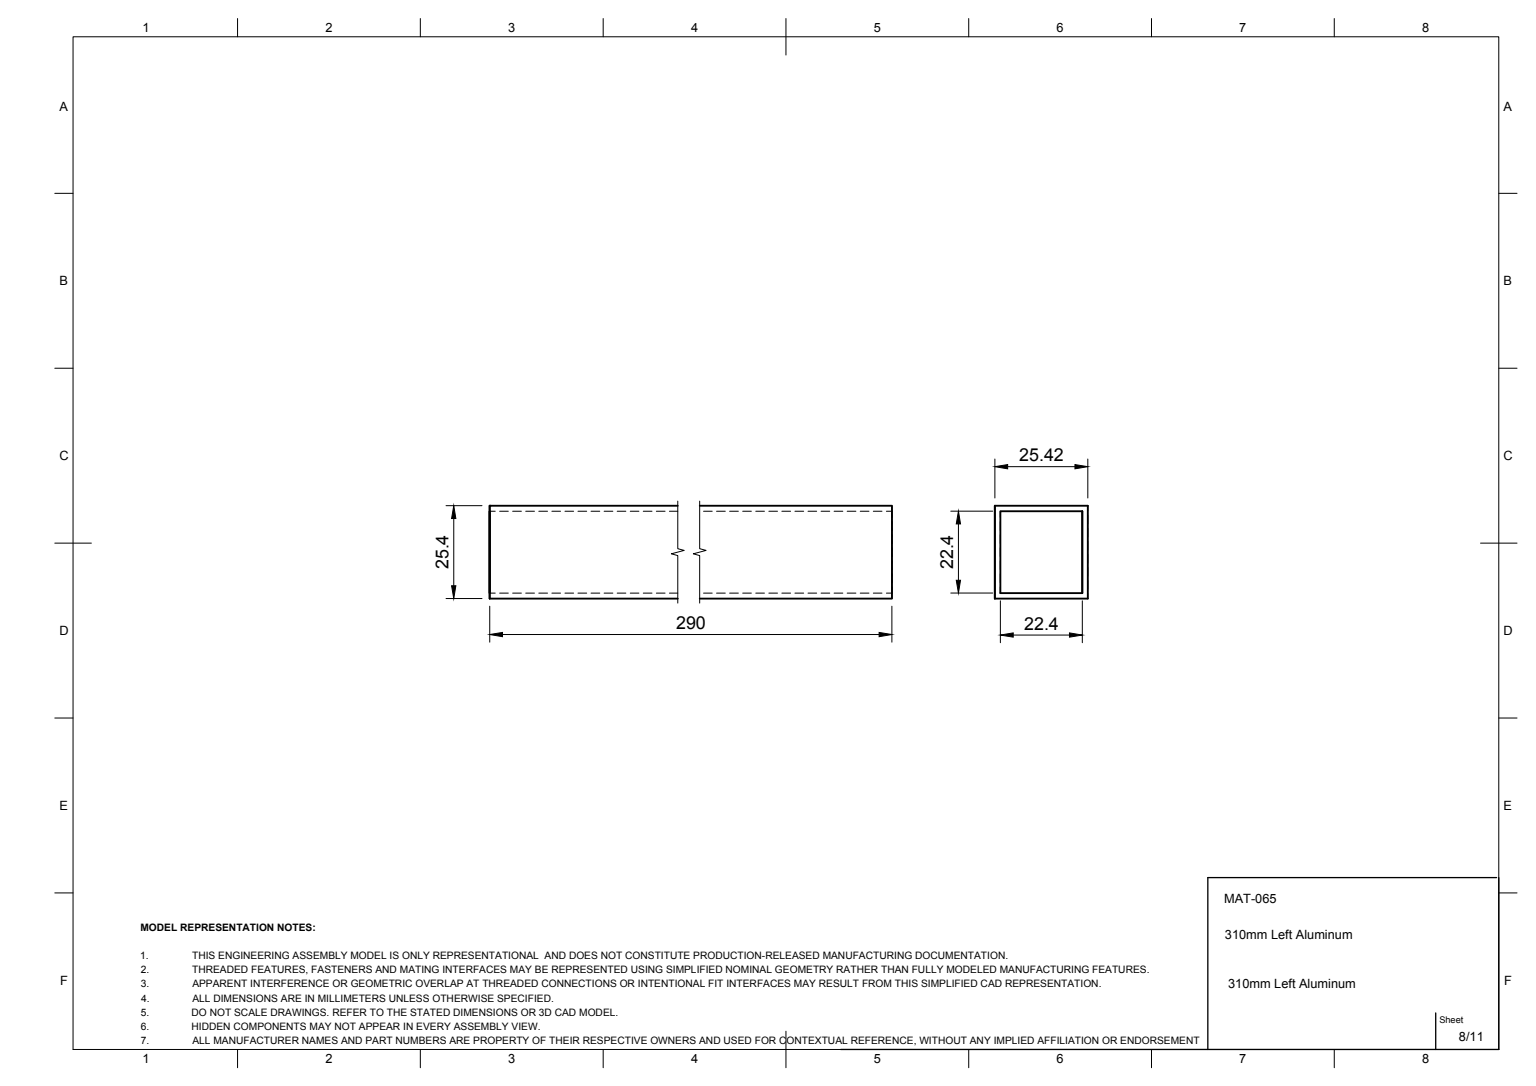
ISO-10303-21;
HEADER;
/* Generated by software containing ST-Developer
 * from STEP Tools, Inc. (www.steptools.com) 
 */

FILE_DESCRIPTION(
/* description */ (
'CAx-IF Rec.Pracs.---Representation and Presentation of Product Manufa
cturing Information (PMI)---4.0---2014-10-13'),
/* implementation_level */ '2;1');

FILE_NAME(
/* name */ '310mm Left Aluminum.step',
/* time_stamp */ '2026-11-15T23:28:27-08:00',
/* author */ (''),
/* organization */ (''),
/* preprocessor_version */ 'ST-DEVELOPER v20.2',
/* originating_system */ 'Autodesk Translation Framework v15.17.0.0',
/* authorisation */ '');

FILE_SCHEMA (('AUTOMOTIVE_DESIGN { 1 0 10303 214 3 1 1 }'));
ENDSEC;

DATA;
#10=MECHANICAL_DESIGN_GEOMETRIC_PRESENTATION_REPRESENTATION('',(#193),#7756);
#175=SHAPE_REPRESENTATION_RELATIONSHIP('SRR','None',#7823,#184);
#184=ADVANCED_BREP_SHAPE_REPRESENTATION('',(#202),#7751);
#193=STYLED_ITEM('',(#7877),#202);
#202=MANIFOLD_SOLID_BREP('Body1',#4630);
#405=FACE_BOUND('',#775,.T.);
#406=FACE_BOUND('',#777,.T.);
#506=FACE_OUTER_BOUND('',#766,.T.);
#507=FACE_OUTER_BOUND('',#767,.T.);
#508=FACE_OUTER_BOUND('',#768,.T.);
#509=FACE_OUTER_BOUND('',#769,.T.);
#510=FACE_OUTER_BOUND('',#770,.T.);
#511=FACE_OUTER_BOUND('',#771,.T.);
#512=FACE_OUTER_BOUND('',#772,.T.);
#513=FACE_OUTER_BOUND('',#773,.T.);
#514=FACE_OUTER_BOUND('',#774,.T.);
#515=FACE_OUTER_BOUND('',#776,.T.);
#766=EDGE_LOOP('',(#3263,#3264,#3265,#3266));
#767=EDGE_LOOP('',(#3267,#3268,#3269,#3270));
#768=EDGE_LOOP('',(#3271,#3272,#3273,#3274));
#769=EDGE_LOOP('',(#3275,#3276,#3277,#3278));
#770=EDGE_LOOP('',(#3279,#3280,#3281,#3282));
#771=EDGE_LOOP('',(#3283,#3284,#3285,#3286));
#772=EDGE_LOOP('',(#3287,#3288,#3289,#3290));
#773=EDGE_LOOP('',(#3291,#3292,#3293,#3294));
#774=EDGE_LOOP('',(#3295,#3296,#3297,#3298));
#775=EDGE_LOOP('',(#3299,#3300,#3301,#3302));
#776=EDGE_LOOP('',(#3303,#3304,#3305,#3306));
#777=EDGE_LOOP('',(#3307,#3308,#3309,#3310));
#1101=LINE('',#6707,#1594);
#1102=LINE('',#6709,#1595);
#1103=LINE('',#6711,#1596);
#1104=LINE('',#6712,#1597);
#1105=LINE('',#6715,#1598);
#1106=LINE('',#6717,#1599);
#1107=LINE('',#6718,#1600);
#1108=LINE('',#6721,#1601);
#1109=LINE('',#6723,#1602);
#1110=LINE('',#6724,#1603);
#1111=LINE('',#6728,#1604);
#1112=LINE('',#6730,#1605);
#1113=LINE('',#6732,#1606);
#1114=LINE('',#6733,#1607);
#1115=LINE('',#6736,#1608);
#1116=LINE('',#6738,#1609);
#1117=LINE('',#6739,#1610);
#1118=LINE('',#6742,#1611);
#1119=LINE('',#6744,#1612);
#1120=LINE('',#6745,#1613);
#1121=LINE('',#6747,#1614);
#1122=LINE('',#6748,#1615);
#1123=LINE('',#6750,#1616);
#1124=LINE('',#6751,#1617);
#1594=VECTOR('',#5415,1.);
#1595=VECTOR('',#5416,1.);
#1596=VECTOR('',#5417,1.);
#1597=VECTOR('',#5418,1.);
#1598=VECTOR('',#5421,1.);
#1599=VECTOR('',#5422,1.);
#1600=VECTOR('',#5423,1.);
#1601=VECTOR('',#5426,1.);
#1602=VECTOR('',#5427,1.);
#1603=VECTOR('',#5428,1.);
#1604=VECTOR('',#5431,1.);
#1605=VECTOR('',#5432,1.);
#1606=VECTOR('',#5433,1.);
#1607=VECTOR('',#5434,1.);
#1608=VECTOR('',#5437,1.);
#1609=VECTOR('',#5438,1.);
#1610=VECTOR('',#5439,1.);
#1611=VECTOR('',#5442,1.);
#1612=VECTOR('',#5443,1.);
#1613=VECTOR('',#5444,1.);
#1614=VECTOR('',#5447,1.);
#1615=VECTOR('',#5448,1.);
#1616=VECTOR('',#5451,1.);
#1617=VECTOR('',#5452,1.);
#2068=VERTEX_POINT('',#6705);
#2069=VERTEX_POINT('',#6706);
#2070=VERTEX_POINT('',#6708);
#2071=VERTEX_POINT('',#6710);
#2072=VERTEX_POINT('',#6714);
#2073=VERTEX_POINT('',#6716);
#2074=VERTEX_POINT('',#6720);
#2075=VERTEX_POINT('',#6722);
#2076=VERTEX_POINT('',#6726);
#2077=VERTEX_POINT('',#6727);
#2078=VERTEX_POINT('',#6729);
#2079=VERTEX_POINT('',#6731);
#2080=VERTEX_POINT('',#6735);
#2081=VERTEX_POINT('',#6737);
#2082=VERTEX_POINT('',#6741);
#2083=VERTEX_POINT('',#6743);
#2515=EDGE_CURVE('',#2068,#2069,#1101,.T.);
#2516=EDGE_CURVE('',#2070,#2068,#1102,.T.);
#2517=EDGE_CURVE('',#2070,#2071,#1103,.T.);
#2518=EDGE_CURVE('',#2071,#2069,#1104,.T.);
#2519=EDGE_CURVE('',#2068,#2072,#1105,.T.);
#2520=EDGE_CURVE('',#2073,#2072,#1106,.T.);
#2521=EDGE_CURVE('',#2070,#2073,#1107,.T.);
#2522=EDGE_CURVE('',#2072,#2074,#1108,.T.);
#2523=EDGE_CURVE('',#2075,#2074,#1109,.T.);
#2524=EDGE_CURVE('',#2073,#2075,#1110,.T.);
#2525=EDGE_CURVE('',#2076,#2077,#1111,.T.);
#2526=EDGE_CURVE('',#2078,#2076,#1112,.T.);
#2527=EDGE_CURVE('',#2078,#2079,#1113,.T.);
#2528=EDGE_CURVE('',#2079,#2077,#1114,.T.);
#2529=EDGE_CURVE('',#2076,#2080,#1115,.T.);
#2530=EDGE_CURVE('',#2081,#2080,#1116,.T.);
#2531=EDGE_CURVE('',#2078,#2081,#1117,.T.);
#2532=EDGE_CURVE('',#2080,#2082,#1118,.T.);
#2533=EDGE_CURVE('',#2083,#2082,#1119,.T.);
#2534=EDGE_CURVE('',#2081,#2083,#1120,.T.);
#2535=EDGE_CURVE('',#2077,#2082,#1121,.T.);
#2536=EDGE_CURVE('',#2079,#2083,#1122,.T.);
#2537=EDGE_CURVE('',#2069,#2074,#1123,.T.);
#2538=EDGE_CURVE('',#2071,#2075,#1124,.T.);
#3263=ORIENTED_EDGE('',*,*,#2515,.F.);
#3264=ORIENTED_EDGE('',*,*,#2516,.F.);
#3265=ORIENTED_EDGE('',*,*,#2517,.T.);
#3266=ORIENTED_EDGE('',*,*,#2518,.T.);
#3267=ORIENTED_EDGE('',*,*,#2519,.T.);
#3268=ORIENTED_EDGE('',*,*,#2520,.F.);
#3269=ORIENTED_EDGE('',*,*,#2521,.F.);
#3270=ORIENTED_EDGE('',*,*,#2516,.T.);
#3271=ORIENTED_EDGE('',*,*,#2522,.T.);
#3272=ORIENTED_EDGE('',*,*,#2523,.F.);
#3273=ORIENTED_EDGE('',*,*,#2524,.F.);
#3274=ORIENTED_EDGE('',*,*,#2520,.T.);
#3275=ORIENTED_EDGE('',*,*,#2525,.F.);
#3276=ORIENTED_EDGE('',*,*,#2526,.F.);
#3277=ORIENTED_EDGE('',*,*,#2527,.T.);
#3278=ORIENTED_EDGE('',*,*,#2528,.T.);
#3279=ORIENTED_EDGE('',*,*,#2529,.T.);
#3280=ORIENTED_EDGE('',*,*,#2530,.F.);
#3281=ORIENTED_EDGE('',*,*,#2531,.F.);
#3282=ORIENTED_EDGE('',*,*,#2526,.T.);
#3283=ORIENTED_EDGE('',*,*,#2532,.T.);
#3284=ORIENTED_EDGE('',*,*,#2533,.F.);
#3285=ORIENTED_EDGE('',*,*,#2534,.F.);
#3286=ORIENTED_EDGE('',*,*,#2530,.T.);
#3287=ORIENTED_EDGE('',*,*,#2535,.F.);
#3288=ORIENTED_EDGE('',*,*,#2528,.F.);
#3289=ORIENTED_EDGE('',*,*,#2536,.T.);
#3290=ORIENTED_EDGE('',*,*,#2533,.T.);
#3291=ORIENTED_EDGE('',*,*,#2537,.F.);
#3292=ORIENTED_EDGE('',*,*,#2518,.F.);
#3293=ORIENTED_EDGE('',*,*,#2538,.T.);
#3294=ORIENTED_EDGE('',*,*,#2523,.T.);
#3295=ORIENTED_EDGE('',*,*,#2517,.F.);
#3296=ORIENTED_EDGE('',*,*,#2521,.T.);
#3297=ORIENTED_EDGE('',*,*,#2524,.T.);
#3298=ORIENTED_EDGE('',*,*,#2538,.F.);
#3299=ORIENTED_EDGE('',*,*,#2527,.F.);
#3300=ORIENTED_EDGE('',*,*,#2531,.T.);
#3301=ORIENTED_EDGE('',*,*,#2534,.T.);
#3302=ORIENTED_EDGE('',*,*,#2536,.F.);
#3303=ORIENTED_EDGE('',*,*,#2515,.T.);
#3304=ORIENTED_EDGE('',*,*,#2537,.T.);
#3305=ORIENTED_EDGE('',*,*,#2522,.F.);
#3306=ORIENTED_EDGE('',*,*,#2519,.F.);
#3307=ORIENTED_EDGE('',*,*,#2525,.T.);
#3308=ORIENTED_EDGE('',*,*,#2535,.T.);
#3309=ORIENTED_EDGE('',*,*,#2532,.F.);
#3310=ORIENTED_EDGE('',*,*,#2529,.F.);
#4260=PLANE('',#4821);
#4261=PLANE('',#4822);
#4262=PLANE('',#4823);
#4263=PLANE('',#4824);
#4264=PLANE('',#4825);
#4265=PLANE('',#4826);
#4266=PLANE('',#4827);
#4267=PLANE('',#4828);
#4268=PLANE('',#4829);
#4269=PLANE('',#4830);
#4447=ADVANCED_FACE('',(#506),#4260,.T.);
#4448=ADVANCED_FACE('',(#507),#4261,.F.);
#4449=ADVANCED_FACE('',(#508),#4262,.F.);
#4450=ADVANCED_FACE('',(#509),#4263,.T.);
#4451=ADVANCED_FACE('',(#510),#4264,.F.);
#4452=ADVANCED_FACE('',(#511),#4265,.F.);
#4453=ADVANCED_FACE('',(#512),#4266,.T.);
#4454=ADVANCED_FACE('',(#513),#4267,.T.);
#4455=ADVANCED_FACE('',(#514,#405),#4268,.T.);
#4456=ADVANCED_FACE('',(#515,#406),#4269,.F.);
#4630=CLOSED_SHELL('',(#4447,#4448,#4449,#4450,#4451,#4452,#4453,#4454,
#4455,#4456));
#4820=AXIS2_PLACEMENT_3D('',#6703,#5411,#5412);
#4821=AXIS2_PLACEMENT_3D('',#6704,#5413,#5414);
#4822=AXIS2_PLACEMENT_3D('',#6713,#5419,#5420);
#4823=AXIS2_PLACEMENT_3D('',#6719,#5424,#5425);
#4824=AXIS2_PLACEMENT_3D('',#6725,#5429,#5430);
#4825=AXIS2_PLACEMENT_3D('',#6734,#5435,#5436);
#4826=AXIS2_PLACEMENT_3D('',#6740,#5440,#5441);
#4827=AXIS2_PLACEMENT_3D('',#6746,#5445,#5446);
#4828=AXIS2_PLACEMENT_3D('',#6749,#5449,#5450);
#4829=AXIS2_PLACEMENT_3D('',#6752,#5453,#5454);
#4830=AXIS2_PLACEMENT_3D('',#6753,#5455,#5456);
#5411=DIRECTION('axis',(0.,0.,1.));
#5412=DIRECTION('refdir',(1.,0.,0.));
#5413=DIRECTION('center_axis',(0.,1.,0.));
#5414=DIRECTION('ref_axis',(0.,0.,1.));
#5415=DIRECTION('',(1.,0.,0.));
#5416=DIRECTION('',(0.,0.,-1.));
#5417=DIRECTION('',(1.,0.,0.));
#5418=DIRECTION('',(0.,0.,-1.));
#5419=DIRECTION('center_axis',(1.,0.,0.));
#5420=DIRECTION('ref_axis',(0.,0.,-1.));
#5421=DIRECTION('',(0.,-1.,0.));
#5422=DIRECTION('',(0.,0.,-1.));
#5423=DIRECTION('',(0.,-1.,0.));
#5424=DIRECTION('center_axis',(0.,1.,0.));
#5425=DIRECTION('ref_axis',(0.,0.,1.));
#5426=DIRECTION('',(1.,0.,0.));
#5427=DIRECTION('',(0.,0.,-1.));
#5428=DIRECTION('',(1.,0.,0.));
#5429=DIRECTION('center_axis',(1.,0.,0.));
#5430=DIRECTION('ref_axis',(0.,0.,-1.));
#5431=DIRECTION('',(0.,-1.,0.));
#5432=DIRECTION('',(0.,0.,-1.));
#5433=DIRECTION('',(0.,-1.,0.));
#5434=DIRECTION('',(0.,0.,-1.));
#5435=DIRECTION('center_axis',(0.,1.,0.));
#5436=DIRECTION('ref_axis',(0.,0.,1.));
#5437=DIRECTION('',(1.,0.,0.));
#5438=DIRECTION('',(0.,0.,-1.));
#5439=DIRECTION('',(1.,0.,0.));
#5440=DIRECTION('center_axis',(1.,0.,0.));
#5441=DIRECTION('ref_axis',(0.,0.,-1.));
#5442=DIRECTION('',(0.,-1.,0.));
#5443=DIRECTION('',(0.,0.,-1.));
#5444=DIRECTION('',(0.,-1.,0.));
#5445=DIRECTION('center_axis',(0.,1.,0.));
#5446=DIRECTION('ref_axis',(0.,0.,1.));
#5447=DIRECTION('',(1.,0.,0.));
#5448=DIRECTION('',(1.,0.,0.));
#5449=DIRECTION('center_axis',(1.,0.,0.));
#5450=DIRECTION('ref_axis',(0.,0.,-1.));
#5451=DIRECTION('',(0.,-1.,0.));
#5452=DIRECTION('',(0.,-1.,0.));
#5453=DIRECTION('center_axis',(0.,0.,1.));
#5454=DIRECTION('ref_axis',(1.,0.,0.));
#5455=DIRECTION('center_axis',(0.,0.,1.));
#5456=DIRECTION('ref_axis',(1.,0.,0.));
#6703=CARTESIAN_POINT('',(0.,0.,0.));
#6704=CARTESIAN_POINT('Origin',(-0.0489786583930254,0.0564453285901962,
0.29));
#6705=CARTESIAN_POINT('',(-0.0616786583930254,0.0564453285901962,0.));
#6706=CARTESIAN_POINT('',(-0.0362786583930254,0.0564453285901962,0.));
#6707=CARTESIAN_POINT('',(-0.0489786583930254,0.0564453285901962,0.));
#6708=CARTESIAN_POINT('',(-0.0616786583930254,0.0564453285901962,0.29));
#6709=CARTESIAN_POINT('',(-0.0616786583930254,0.0564453285901962,0.29));
#6710=CARTESIAN_POINT('',(-0.0362786583930254,0.0564453285901962,0.29));
#6711=CARTESIAN_POINT('',(-0.0489786583930254,0.0564453285901962,0.29));
#6712=CARTESIAN_POINT('',(-0.0362786583930254,0.0564453285901962,0.29));
#6713=CARTESIAN_POINT('Origin',(-0.0616786583930254,0.0437453285901962,
0.29));
#6714=CARTESIAN_POINT('',(-0.0616786583930254,0.0310453285901962,0.));
#6715=CARTESIAN_POINT('',(-0.0616786583930254,0.0437453285901962,0.));
#6716=CARTESIAN_POINT('',(-0.0616786583930254,0.0310453285901962,0.29));
#6717=CARTESIAN_POINT('',(-0.0616786583930254,0.0310453285901962,0.29));
#6718=CARTESIAN_POINT('',(-0.0616786583930254,0.0437453285901962,0.29));
#6719=CARTESIAN_POINT('Origin',(-0.0489786583930254,0.0310453285901962,
0.29));
#6720=CARTESIAN_POINT('',(-0.0362786583930254,0.0310453285901962,0.));
#6721=CARTESIAN_POINT('',(-0.0489786583930254,0.0310453285901962,0.));
#6722=CARTESIAN_POINT('',(-0.0362786583930254,0.0310453285901962,0.29));
#6723=CARTESIAN_POINT('',(-0.0362786583930254,0.0310453285901962,0.29));
#6724=CARTESIAN_POINT('',(-0.0489786583930254,0.0310453285901962,0.29));
#6725=CARTESIAN_POINT('Origin',(-0.0601786583930254,0.0437453285901962,
0.29));
#6726=CARTESIAN_POINT('',(-0.0601786583930254,0.0549453285901962,0.));
#6727=CARTESIAN_POINT('',(-0.0601786583930254,0.0325453285901962,0.));
#6728=CARTESIAN_POINT('',(-0.0601786583930254,0.0437453285901962,0.));
#6729=CARTESIAN_POINT('',(-0.0601786583930254,0.0549453285901962,0.29));
#6730=CARTESIAN_POINT('',(-0.0601786583930254,0.0549453285901962,0.29));
#6731=CARTESIAN_POINT('',(-0.0601786583930254,0.0325453285901962,0.29));
#6732=CARTESIAN_POINT('',(-0.0601786583930254,0.0437453285901962,0.29));
#6733=CARTESIAN_POINT('',(-0.0601786583930254,0.0325453285901962,0.29));
#6734=CARTESIAN_POINT('Origin',(-0.0489786583930254,0.0549453285901962,
0.29));
#6735=CARTESIAN_POINT('',(-0.0377786583930254,0.0549453285901962,0.));
#6736=CARTESIAN_POINT('',(-0.0489786583930254,0.0549453285901962,0.));
#6737=CARTESIAN_POINT('',(-0.0377786583930254,0.0549453285901962,0.29));
#6738=CARTESIAN_POINT('',(-0.0377786583930254,0.0549453285901962,0.29));
#6739=CARTESIAN_POINT('',(-0.0489786583930254,0.0549453285901962,0.29));
#6740=CARTESIAN_POINT('Origin',(-0.0377786583930254,0.0437453285901962,
0.29));
#6741=CARTESIAN_POINT('',(-0.0377786583930254,0.0325453285901962,0.));
#6742=CARTESIAN_POINT('',(-0.0377786583930254,0.0437453285901962,0.));
#6743=CARTESIAN_POINT('',(-0.0377786583930254,0.0325453285901962,0.29));
#6744=CARTESIAN_POINT('',(-0.0377786583930254,0.0325453285901962,0.29));
#6745=CARTESIAN_POINT('',(-0.0377786583930254,0.0437453285901962,0.29));
#6746=CARTESIAN_POINT('Origin',(-0.0489786583930254,0.0325453285901962,
0.29));
#6747=CARTESIAN_POINT('',(-0.0489786583930254,0.0325453285901962,0.));
#6748=CARTESIAN_POINT('',(-0.0489786583930254,0.0325453285901962,0.29));
#6749=CARTESIAN_POINT('Origin',(-0.0362786583930254,0.0437453285901962,
0.29));
#6750=CARTESIAN_POINT('',(-0.0362786583930254,0.0437453285901962,0.));
#6751=CARTESIAN_POINT('',(-0.0362786583930254,0.0437453285901962,0.29));
#6752=CARTESIAN_POINT('Origin',(-0.0489786583930254,0.0437453285901962,
0.29));
#6753=CARTESIAN_POINT('Origin',(-0.0489786583930254,0.0437453285901962,
0.));
#7740=UNCERTAINTY_MEASURE_WITH_UNIT(LENGTH_MEASURE(1.E-5),#7757,
'DISTANCE_ACCURACY_VALUE',
'Maximum model space distance between geometric entities at asserted c
onnectivities');
#7745=UNCERTAINTY_MEASURE_WITH_UNIT(LENGTH_MEASURE(1.E-5),#7757,
'DISTANCE_ACCURACY_VALUE',
'Maximum model space distance between geometric entities at asserted c
onnectivities');
#7751=(
GEOMETRIC_REPRESENTATION_CONTEXT(3)
GLOBAL_UNCERTAINTY_ASSIGNED_CONTEXT((#7740))
GLOBAL_UNIT_ASSIGNED_CONTEXT((#7757,#7758,#7759))
REPRESENTATION_CONTEXT('','3D')
);
#7756=(
GEOMETRIC_REPRESENTATION_CONTEXT(3)
GLOBAL_UNCERTAINTY_ASSIGNED_CONTEXT((#7745))
GLOBAL_UNIT_ASSIGNED_CONTEXT((#7757,#7758,#7759))
REPRESENTATION_CONTEXT('','3D')
);
#7757=(
LENGTH_UNIT()
NAMED_UNIT(*)
SI_UNIT($,.METRE.)
);
#7758=(
NAMED_UNIT(*)
PLANE_ANGLE_UNIT()
SI_UNIT($,.RADIAN.)
);
#7759=(
NAMED_UNIT(*)
SI_UNIT($,.STERADIAN.)
SOLID_ANGLE_UNIT()
);
#7765=SHAPE_DEFINITION_REPRESENTATION(#7775,#7823);
#7775=PRODUCT_DEFINITION_SHAPE('',$,#7834);
#7823=SHAPE_REPRESENTATION('',(#4820),#7751);
#7828=PRODUCT_DEFINITION_CONTEXT('part definition',#7860,'design');
#7834=PRODUCT_DEFINITION('310mm Left Aluminum','310mm Left Aluminum',#7844,
#7828);
#7844=PRODUCT_DEFINITION_FORMATION('',$,#7867);
#7860=APPLICATION_CONTEXT(
'Core Data for Automotive Mechanical Design Process');
#7861=PRODUCT_CONTEXT('part definition',#7860,'mechanical');
#7867=PRODUCT('310mm Left Aluminum','310mm Left Aluminum',
'LEGAL AND USAGE DISCLAIMER: this Data/Model is provided \X2\201C\X0\A
S IS\X2\201D\X0\ for informational and representational only. It is a 
geometric approximation and is NOT engineered, certified, or guarantee
d for dimensional accuracy, exact tolerances, or production-level prec
ision. Vendor disclaims all implied warranties including fitness for a
 particular purpose. DO NOT USE FOR DIRECT PHYSICAL MANUFACTURING, AUT
OMATED PRODUCTION, OR SAFETY-CRITICAL SYSTEMS without independent engi
neering verification and resolution of any design discrepancies.',(#7861));
#7877=PRESENTATION_STYLE_ASSIGNMENT((#7884));
#7884=SURFACE_STYLE_USAGE(.BOTH.,#7891);
#7891=SURFACE_SIDE_STYLE('',(#7898));
#7898=SURFACE_STYLE_FILL_AREA(#7905);
#7905=FILL_AREA_STYLE('Opaque(89,149,218)',(#7912));
#7912=FILL_AREA_STYLE_COLOUR('Opaque(89,149,218)',#7919);
#7919=COLOUR_RGB('Opaque(89,149,218)',0.349019607843137,0.584313725490196,
0.854901960784314);
ENDSEC;
END-ISO-10303-21;
